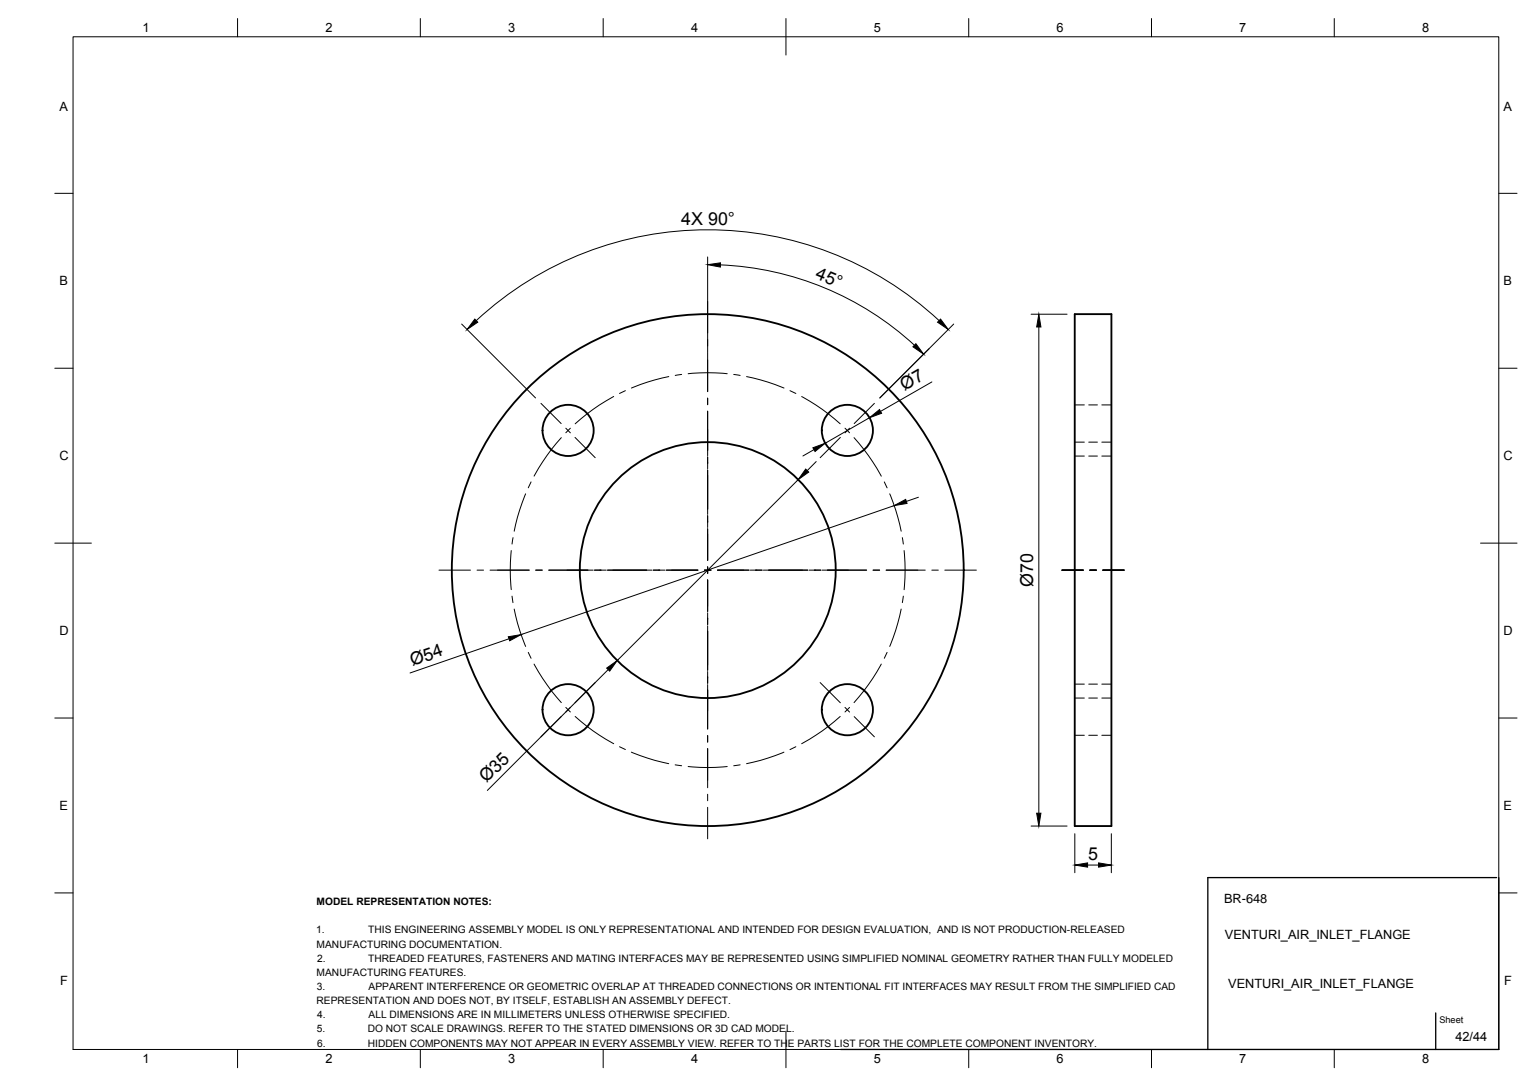
ISO-10303-21;
HEADER;
FILE_DESCRIPTION((''),'2;1');
FILE_NAME('VENTURI_AIR_INLET_FLANGE.step','2026-10-01T22:05:39-07:00',(''),(''),'','','');
FILE_SCHEMA (('AUTOMOTIVE_DESIGN { 1 0 10303 214 3 1 1 }'));
ENDSEC;
DATA;
#10=MECHANICAL_DESIGN_GEOMETRIC_PRESENTATION_REPRESENTATION('',(#638),#24628);
#554=SHAPE_REPRESENTATION_RELATIONSHIP('SRR','None',#24828,#596) ;
#596=ADVANCED_BREP_SHAPE_REPRESENTATION('',(#677),#24618) ;
#638=STYLED_ITEM('',(#25031),#677) ;
#677=MANIFOLD_SOLID_BREP('VENTURI_AIR_INLET_FLANGE',#13180) ;
#914=FACE_BOUND('',#4643,.T.) ;
#915=FACE_BOUND('',#4644,.T.) ;
#916=FACE_BOUND('',#4645,.T.) ;
#917=FACE_BOUND('',#4646,.T.) ;
#918=FACE_BOUND('',#4647,.T.) ;
#919=FACE_BOUND('',#4649,.T.) ;
#920=FACE_BOUND('',#4650,.T.) ;
#921=FACE_BOUND('',#4651,.T.) ;
#922=FACE_BOUND('',#4652,.T.) ;
#923=FACE_BOUND('',#4653,.T.) ;
#1724=LINE('',#24110,#2560) ;
#1725=LINE('',#24116,#2561) ;
#1726=LINE('',#24122,#2562) ;
#1727=LINE('',#24128,#2563) ;
#1728=LINE('',#24134,#2564) ;
#1729=LINE('',#24140,#2565) ;
#2560=VECTOR('',#19259,0.35) ;
#2561=VECTOR('',#19266,0.35) ;
#2562=VECTOR('',#19273,0.35) ;
#2563=VECTOR('',#19280,0.35) ;
#2564=VECTOR('',#19287,1.75) ;
#2565=VECTOR('',#19294,3.5) ;
#2926=CYLINDRICAL_SURFACE('',#15223,0.35) ;
#2927=CYLINDRICAL_SURFACE('',#15226,0.35) ;
#2928=CYLINDRICAL_SURFACE('',#15229,0.35) ;
#2929=CYLINDRICAL_SURFACE('',#15232,0.35) ;
#2930=CYLINDRICAL_SURFACE('',#15235,1.75) ;
#2931=CYLINDRICAL_SURFACE('',#15238,3.5) ;
#3641=FACE_OUTER_BOUND('',#4636,.T.) ;
#3642=FACE_OUTER_BOUND('',#4637,.T.) ;
#3643=FACE_OUTER_BOUND('',#4638,.T.) ;
#3644=FACE_OUTER_BOUND('',#4639,.T.) ;
#3645=FACE_OUTER_BOUND('',#4640,.T.) ;
#3646=FACE_OUTER_BOUND('',#4641,.T.) ;
#3647=FACE_OUTER_BOUND('',#4642,.T.) ;
#3648=FACE_OUTER_BOUND('',#4648,.T.) ;
#4636=EDGE_LOOP('',(#11665,#11666,#11667,#11668)) ;
#4637=EDGE_LOOP('',(#11669,#11670,#11671,#11672)) ;
#4638=EDGE_LOOP('',(#11673,#11674,#11675,#11676)) ;
#4639=EDGE_LOOP('',(#11677,#11678,#11679,#11680)) ;
#4640=EDGE_LOOP('',(#11681,#11682,#11683,#11684)) ;
#4641=EDGE_LOOP('',(#11685,#11686,#11687,#11688)) ;
#4642=EDGE_LOOP('',(#11689)) ;
#4643=EDGE_LOOP('',(#11690)) ;
#4644=EDGE_LOOP('',(#11691)) ;
#4645=EDGE_LOOP('',(#11692)) ;
#4646=EDGE_LOOP('',(#11693)) ;
#4647=EDGE_LOOP('',(#11694)) ;
#4648=EDGE_LOOP('',(#11695)) ;
#4649=EDGE_LOOP('',(#11696)) ;
#4650=EDGE_LOOP('',(#11697)) ;
#4651=EDGE_LOOP('',(#11698)) ;
#4652=EDGE_LOOP('',(#11699)) ;
#4653=EDGE_LOOP('',(#11700)) ;
#5487=CIRCLE('',#15224,0.35) ;
#5488=CIRCLE('',#15225,0.35) ;
#5489=CIRCLE('',#15227,0.35) ;
#5490=CIRCLE('',#15228,0.35) ;
#5491=CIRCLE('',#15230,0.35) ;
#5492=CIRCLE('',#15231,0.35) ;
#5493=CIRCLE('',#15233,0.35) ;
#5494=CIRCLE('',#15234,0.35) ;
#5495=CIRCLE('',#15236,1.75) ;
#5496=CIRCLE('',#15237,1.75) ;
#5497=CIRCLE('',#15239,3.5) ;
#5498=CIRCLE('',#15240,3.5) ;
#6623=VERTEX_POINT('',#24107) ;
#6624=VERTEX_POINT('',#24109) ;
#6625=VERTEX_POINT('',#24113) ;
#6626=VERTEX_POINT('',#24115) ;
#6627=VERTEX_POINT('',#24119) ;
#6628=VERTEX_POINT('',#24121) ;
#6629=VERTEX_POINT('',#24125) ;
#6630=VERTEX_POINT('',#24127) ;
#6631=VERTEX_POINT('',#24131) ;
#6632=VERTEX_POINT('',#24133) ;
#6633=VERTEX_POINT('',#24137) ;
#6634=VERTEX_POINT('',#24139) ;
#8322=EDGE_CURVE('',#6623,#6623,#5487,.T.) ;
#8323=EDGE_CURVE('',#6623,#6624,#1724,.T.) ;
#8324=EDGE_CURVE('',#6624,#6624,#5488,.T.) ;
#8325=EDGE_CURVE('',#6625,#6625,#5489,.T.) ;
#8326=EDGE_CURVE('',#6625,#6626,#1725,.T.) ;
#8327=EDGE_CURVE('',#6626,#6626,#5490,.T.) ;
#8328=EDGE_CURVE('',#6627,#6627,#5491,.T.) ;
#8329=EDGE_CURVE('',#6627,#6628,#1726,.T.) ;
#8330=EDGE_CURVE('',#6628,#6628,#5492,.T.) ;
#8331=EDGE_CURVE('',#6629,#6629,#5493,.T.) ;
#8332=EDGE_CURVE('',#6629,#6630,#1727,.T.) ;
#8333=EDGE_CURVE('',#6630,#6630,#5494,.T.) ;
#8334=EDGE_CURVE('',#6631,#6631,#5495,.T.) ;
#8335=EDGE_CURVE('',#6631,#6632,#1728,.T.) ;
#8336=EDGE_CURVE('',#6632,#6632,#5496,.T.) ;
#8337=EDGE_CURVE('',#6633,#6633,#5497,.T.) ;
#8338=EDGE_CURVE('',#6633,#6634,#1729,.T.) ;
#8339=EDGE_CURVE('',#6634,#6634,#5498,.T.) ;
#11665=ORIENTED_EDGE('',*,*,#8322,.F.) ;
#11666=ORIENTED_EDGE('',*,*,#8323,.T.) ;
#11667=ORIENTED_EDGE('',*,*,#8324,.F.) ;
#11668=ORIENTED_EDGE('',*,*,#8323,.F.) ;
#11669=ORIENTED_EDGE('',*,*,#8325,.F.) ;
#11670=ORIENTED_EDGE('',*,*,#8326,.T.) ;
#11671=ORIENTED_EDGE('',*,*,#8327,.F.) ;
#11672=ORIENTED_EDGE('',*,*,#8326,.F.) ;
#11673=ORIENTED_EDGE('',*,*,#8328,.F.) ;
#11674=ORIENTED_EDGE('',*,*,#8329,.T.) ;
#11675=ORIENTED_EDGE('',*,*,#8330,.F.) ;
#11676=ORIENTED_EDGE('',*,*,#8329,.F.) ;
#11677=ORIENTED_EDGE('',*,*,#8331,.F.) ;
#11678=ORIENTED_EDGE('',*,*,#8332,.T.) ;
#11679=ORIENTED_EDGE('',*,*,#8333,.F.) ;
#11680=ORIENTED_EDGE('',*,*,#8332,.F.) ;
#11681=ORIENTED_EDGE('',*,*,#8334,.F.) ;
#11682=ORIENTED_EDGE('',*,*,#8335,.T.) ;
#11683=ORIENTED_EDGE('',*,*,#8336,.F.) ;
#11684=ORIENTED_EDGE('',*,*,#8335,.F.) ;
#11685=ORIENTED_EDGE('',*,*,#8337,.F.) ;
#11686=ORIENTED_EDGE('',*,*,#8338,.T.) ;
#11687=ORIENTED_EDGE('',*,*,#8339,.F.) ;
#11688=ORIENTED_EDGE('',*,*,#8338,.F.) ;
#11689=ORIENTED_EDGE('',*,*,#8339,.T.) ;
#11690=ORIENTED_EDGE('',*,*,#8322,.T.) ;
#11691=ORIENTED_EDGE('',*,*,#8325,.T.) ;
#11692=ORIENTED_EDGE('',*,*,#8328,.T.) ;
#11693=ORIENTED_EDGE('',*,*,#8331,.T.) ;
#11694=ORIENTED_EDGE('',*,*,#8334,.T.) ;
#11695=ORIENTED_EDGE('',*,*,#8337,.T.) ;
#11696=ORIENTED_EDGE('',*,*,#8324,.T.) ;
#11697=ORIENTED_EDGE('',*,*,#8327,.T.) ;
#11698=ORIENTED_EDGE('',*,*,#8330,.T.) ;
#11699=ORIENTED_EDGE('',*,*,#8333,.T.) ;
#11700=ORIENTED_EDGE('',*,*,#8336,.T.) ;
#12295=PLANE('',#15241) ;
#12296=PLANE('',#15242) ;
#13036=ADVANCED_FACE('',(#3641),#2926,.F.) ;
#13037=ADVANCED_FACE('',(#3642),#2927,.F.) ;
#13038=ADVANCED_FACE('',(#3643),#2928,.F.) ;
#13039=ADVANCED_FACE('',(#3644),#2929,.F.) ;
#13040=ADVANCED_FACE('',(#3645),#2930,.F.) ;
#13041=ADVANCED_FACE('',(#3646),#2931,.T.) ;
#13042=ADVANCED_FACE('',(#3647,#914,#915,#916,#917,#918),#12295,.T.) ;
#13043=ADVANCED_FACE('',(#3648,#919,#920,#921,#922,#923),#12296,.T.) ;
#13180=CLOSED_SHELL('',(#13036,#13037,#13038,#13039,#13040,#13041,#13042,
#13043)) ;
#15222=AXIS2_PLACEMENT_3D('',#24105,#19253,#19254) ;
#15223=AXIS2_PLACEMENT_3D('',#24106,#19255,#19256) ;
#15224=AXIS2_PLACEMENT_3D('',#24108,#19257,#19258) ;
#15225=AXIS2_PLACEMENT_3D('',#24111,#19260,#19261) ;
#15226=AXIS2_PLACEMENT_3D('',#24112,#19262,#19263) ;
#15227=AXIS2_PLACEMENT_3D('',#24114,#19264,#19265) ;
#15228=AXIS2_PLACEMENT_3D('',#24117,#19267,#19268) ;
#15229=AXIS2_PLACEMENT_3D('',#24118,#19269,#19270) ;
#15230=AXIS2_PLACEMENT_3D('',#24120,#19271,#19272) ;
#15231=AXIS2_PLACEMENT_3D('',#24123,#19274,#19275) ;
#15232=AXIS2_PLACEMENT_3D('',#24124,#19276,#19277) ;
#15233=AXIS2_PLACEMENT_3D('',#24126,#19278,#19279) ;
#15234=AXIS2_PLACEMENT_3D('',#24129,#19281,#19282) ;
#15235=AXIS2_PLACEMENT_3D('',#24130,#19283,#19284) ;
#15236=AXIS2_PLACEMENT_3D('',#24132,#19285,#19286) ;
#15237=AXIS2_PLACEMENT_3D('',#24135,#19288,#19289) ;
#15238=AXIS2_PLACEMENT_3D('',#24136,#19290,#19291) ;
#15239=AXIS2_PLACEMENT_3D('',#24138,#19292,#19293) ;
#15240=AXIS2_PLACEMENT_3D('',#24141,#19295,#19296) ;
#15241=AXIS2_PLACEMENT_3D('',#24142,#19297,#19298) ;
#15242=AXIS2_PLACEMENT_3D('',#24143,#19299,#19300) ;
#19253=DIRECTION('axis',(0.,0.,1.)) ;
#19254=DIRECTION('refdir',(1.,0.,0.)) ;
#19255=DIRECTION('center_axis',(1.,0.,0.)) ;
#19256=DIRECTION('ref_axis',(0.,0.,-1.)) ;
#19257=DIRECTION('center_axis',(1.,0.,0.)) ;
#19258=DIRECTION('ref_axis',(0.,0.,-1.)) ;
#19259=DIRECTION('',(1.,0.,0.)) ;
#19260=DIRECTION('center_axis',(-1.,0.,0.)) ;
#19261=DIRECTION('ref_axis',(0.,0.,-1.)) ;
#19262=DIRECTION('center_axis',(1.,0.,0.)) ;
#19263=DIRECTION('ref_axis',(0.,0.,-1.)) ;
#19264=DIRECTION('center_axis',(1.,0.,0.)) ;
#19265=DIRECTION('ref_axis',(0.,0.,-1.)) ;
#19266=DIRECTION('',(1.,0.,0.)) ;
#19267=DIRECTION('center_axis',(-1.,0.,0.)) ;
#19268=DIRECTION('ref_axis',(0.,0.,-1.)) ;
#19269=DIRECTION('center_axis',(1.,0.,0.)) ;
#19270=DIRECTION('ref_axis',(0.,0.,-1.)) ;
#19271=DIRECTION('center_axis',(1.,0.,0.)) ;
#19272=DIRECTION('ref_axis',(0.,0.,-1.)) ;
#19273=DIRECTION('',(1.,0.,0.)) ;
#19274=DIRECTION('center_axis',(-1.,0.,0.)) ;
#19275=DIRECTION('ref_axis',(0.,0.,-1.)) ;
#19276=DIRECTION('center_axis',(1.,0.,0.)) ;
#19277=DIRECTION('ref_axis',(0.,0.,-1.)) ;
#19278=DIRECTION('center_axis',(1.,0.,0.)) ;
#19279=DIRECTION('ref_axis',(0.,0.,-1.)) ;
#19280=DIRECTION('',(1.,0.,0.)) ;
#19281=DIRECTION('center_axis',(-1.,0.,0.)) ;
#19282=DIRECTION('ref_axis',(0.,0.,-1.)) ;
#19283=DIRECTION('center_axis',(1.,0.,0.)) ;
#19284=DIRECTION('ref_axis',(0.,0.,-1.)) ;
#19285=DIRECTION('center_axis',(1.,0.,0.)) ;
#19286=DIRECTION('ref_axis',(0.,0.,-1.)) ;
#19287=DIRECTION('',(1.,0.,0.)) ;
#19288=DIRECTION('center_axis',(-1.,0.,0.)) ;
#19289=DIRECTION('ref_axis',(0.,0.,-1.)) ;
#19290=DIRECTION('center_axis',(1.,0.,0.)) ;
#19291=DIRECTION('ref_axis',(0.,0.,-1.)) ;
#19292=DIRECTION('center_axis',(1.,0.,0.)) ;
#19293=DIRECTION('ref_axis',(0.,0.,-1.)) ;
#19294=DIRECTION('',(-1.,0.,0.)) ;
#19295=DIRECTION('center_axis',(-1.,0.,0.)) ;
#19296=DIRECTION('ref_axis',(0.,0.,-1.)) ;
#19297=DIRECTION('center_axis',(-1.,0.,0.)) ;
#19298=DIRECTION('ref_axis',(0.,0.,1.)) ;
#19299=DIRECTION('center_axis',(1.,0.,0.)) ;
#19300=DIRECTION('ref_axis',(0.,0.,-1.)) ;
#24105=CARTESIAN_POINT('',(0.,0.,0.)) ;
#24106=CARTESIAN_POINT('Origin',(-29.75,0.109188309203678,-18.4091883092037)) ;
#24107=CARTESIAN_POINT('',(-30.,0.109188309203678,-18.0591883092037)) ;
#24108=CARTESIAN_POINT('Origin',(-30.,0.109188309203678,-18.4091883092037)) ;
#24109=CARTESIAN_POINT('',(-29.5,0.109188309203678,-18.0591883092037)) ;
#24110=CARTESIAN_POINT('',(-29.75,0.109188309203678,-18.0591883092037)) ;
#24111=CARTESIAN_POINT('Origin',(-29.5,0.109188309203678,-18.4091883092037)) ;
#24112=CARTESIAN_POINT('Origin',(-29.75,-3.70918830920368,-18.4091883092037)) ;
#24113=CARTESIAN_POINT('',(-30.,-3.70918830920368,-18.0591883092037)) ;
#24114=CARTESIAN_POINT('Origin',(-30.,-3.70918830920368,-18.4091883092037)) ;
#24115=CARTESIAN_POINT('',(-29.5,-3.70918830920368,-18.0591883092037)) ;
#24116=CARTESIAN_POINT('',(-29.75,-3.70918830920368,-18.0591883092037)) ;
#24117=CARTESIAN_POINT('Origin',(-29.5,-3.70918830920368,-18.4091883092037)) ;
#24118=CARTESIAN_POINT('Origin',(-29.75,-3.70918830920368,-14.5908116907963)) ;
#24119=CARTESIAN_POINT('',(-30.,-3.70918830920368,-14.2408116907963)) ;
#24120=CARTESIAN_POINT('Origin',(-30.,-3.70918830920368,-14.5908116907963)) ;
#24121=CARTESIAN_POINT('',(-29.5,-3.70918830920368,-14.2408116907963)) ;
#24122=CARTESIAN_POINT('',(-29.75,-3.70918830920368,-14.2408116907963)) ;
#24123=CARTESIAN_POINT('Origin',(-29.5,-3.70918830920368,-14.5908116907963)) ;
#24124=CARTESIAN_POINT('Origin',(-29.75,0.109188309203678,-14.5908116907963)) ;
#24125=CARTESIAN_POINT('',(-30.,0.109188309203678,-14.2408116907963)) ;
#24126=CARTESIAN_POINT('Origin',(-30.,0.109188309203678,-14.5908116907963)) ;
#24127=CARTESIAN_POINT('',(-29.5,0.109188309203679,-14.2408116907963)) ;
#24128=CARTESIAN_POINT('',(-29.75,0.109188309203678,-14.2408116907963)) ;
#24129=CARTESIAN_POINT('Origin',(-29.5,0.109188309203678,-14.5908116907963)) ;
#24130=CARTESIAN_POINT('Origin',(-29.75,-1.8,-16.5)) ;
#24131=CARTESIAN_POINT('',(-30.,-1.8,-14.75)) ;
#24132=CARTESIAN_POINT('Origin',(-30.,-1.8,-16.5)) ;
#24133=CARTESIAN_POINT('',(-29.5,-1.8,-14.75)) ;
#24134=CARTESIAN_POINT('',(-29.75,-1.8,-14.75)) ;
#24135=CARTESIAN_POINT('Origin',(-29.5,-1.8,-16.5)) ;
#24136=CARTESIAN_POINT('Origin',(-29.75,-1.8,-16.5)) ;
#24137=CARTESIAN_POINT('',(-29.5,-1.8,-13.)) ;
#24138=CARTESIAN_POINT('Origin',(-29.5,-1.8,-16.5)) ;
#24139=CARTESIAN_POINT('',(-30.,-1.8,-13.)) ;
#24140=CARTESIAN_POINT('',(-29.75,-1.8,-13.)) ;
#24141=CARTESIAN_POINT('Origin',(-30.,-1.8,-16.5)) ;
#24142=CARTESIAN_POINT('Origin',(-30.,-1.8,-16.5)) ;
#24143=CARTESIAN_POINT('Origin',(-29.5,-1.8,-16.5)) ;
#24570=UNCERTAINTY_MEASURE_WITH_UNIT(LENGTH_MEASURE(0.001),#24629,
'DISTANCE_ACCURACY_VALUE',
'Maximum model space distance between geometric entities at asserted c
onnectivities') ;
#24580=UNCERTAINTY_MEASURE_WITH_UNIT(LENGTH_MEASURE(0.001),#24629,
'DISTANCE_ACCURACY_VALUE',
'Maximum model space distance between geometric entities at asserted c
onnectivities') ;
#24618=(
GEOMETRIC_REPRESENTATION_CONTEXT(3)
GLOBAL_UNCERTAINTY_ASSIGNED_CONTEXT((#24570))
GLOBAL_UNIT_ASSIGNED_CONTEXT((#24629,#24631,#24632))
REPRESENTATION_CONTEXT('','3D')
) ;
#24628=(
GEOMETRIC_REPRESENTATION_CONTEXT(3)
GLOBAL_UNCERTAINTY_ASSIGNED_CONTEXT((#24580))
GLOBAL_UNIT_ASSIGNED_CONTEXT((#24629,#24631,#24632))
REPRESENTATION_CONTEXT('','3D')
) ;
#24629=(
LENGTH_UNIT()
NAMED_UNIT(*)
SI_UNIT(.CENTI.,.METRE.)
) ;
#24631=(
NAMED_UNIT(*)
PLANE_ANGLE_UNIT()
SI_UNIT($,.RADIAN.)
) ;
#24632=(
NAMED_UNIT(*)
SI_UNIT($,.STERADIAN.)
SOLID_ANGLE_UNIT()
) ;
#24670=SHAPE_DEFINITION_REPRESENTATION(#24751,#24828) ;
#24751=PRODUCT_DEFINITION_SHAPE('',$,#24876) ;
#24828=SHAPE_REPRESENTATION('',(#15222),#24618) ;
#24838=PRODUCT_DEFINITION_CONTEXT('part definition',#24981,'design') ;
#24876=PRODUCT_DEFINITION('VENTURI_AIR_INLET_FLANGE',
'VENTURI_AIR_INLET_FLANGE',#24923,#24838) ;
#24923=PRODUCT_DEFINITION_FORMATION('',$,#25020) ;
#24981=APPLICATION_CONTEXT(
'Core Data for Automotive Mechanical Design Process') ;
#24982=PRODUCT_CONTEXT('part definition',#24981,'mechanical') ;
#25020=PRODUCT('VENTURI_AIR_INLET_FLANGE','VENTURI_AIR_INLET_FLANGE',$,(#24982)) ;
#25031=PRESENTATION_STYLE_ASSIGNMENT((#25041)) ;
#25041=SURFACE_STYLE_USAGE(.BOTH.,#25051) ;
#25051=SURFACE_SIDE_STYLE('',(#25061)) ;
#25061=SURFACE_STYLE_FILL_AREA(#25071) ;
#25071=FILL_AREA_STYLE('Aluminum - Satin',(#25081)) ;
#25081=FILL_AREA_STYLE_COLOUR('Aluminum - Satin',#25091) ;
#25091=COLOUR_RGB('Aluminum - Satin', 0.40784314, 0.44705882, 0.49803922) ;
ENDSEC;
END-ISO-10303-21;
